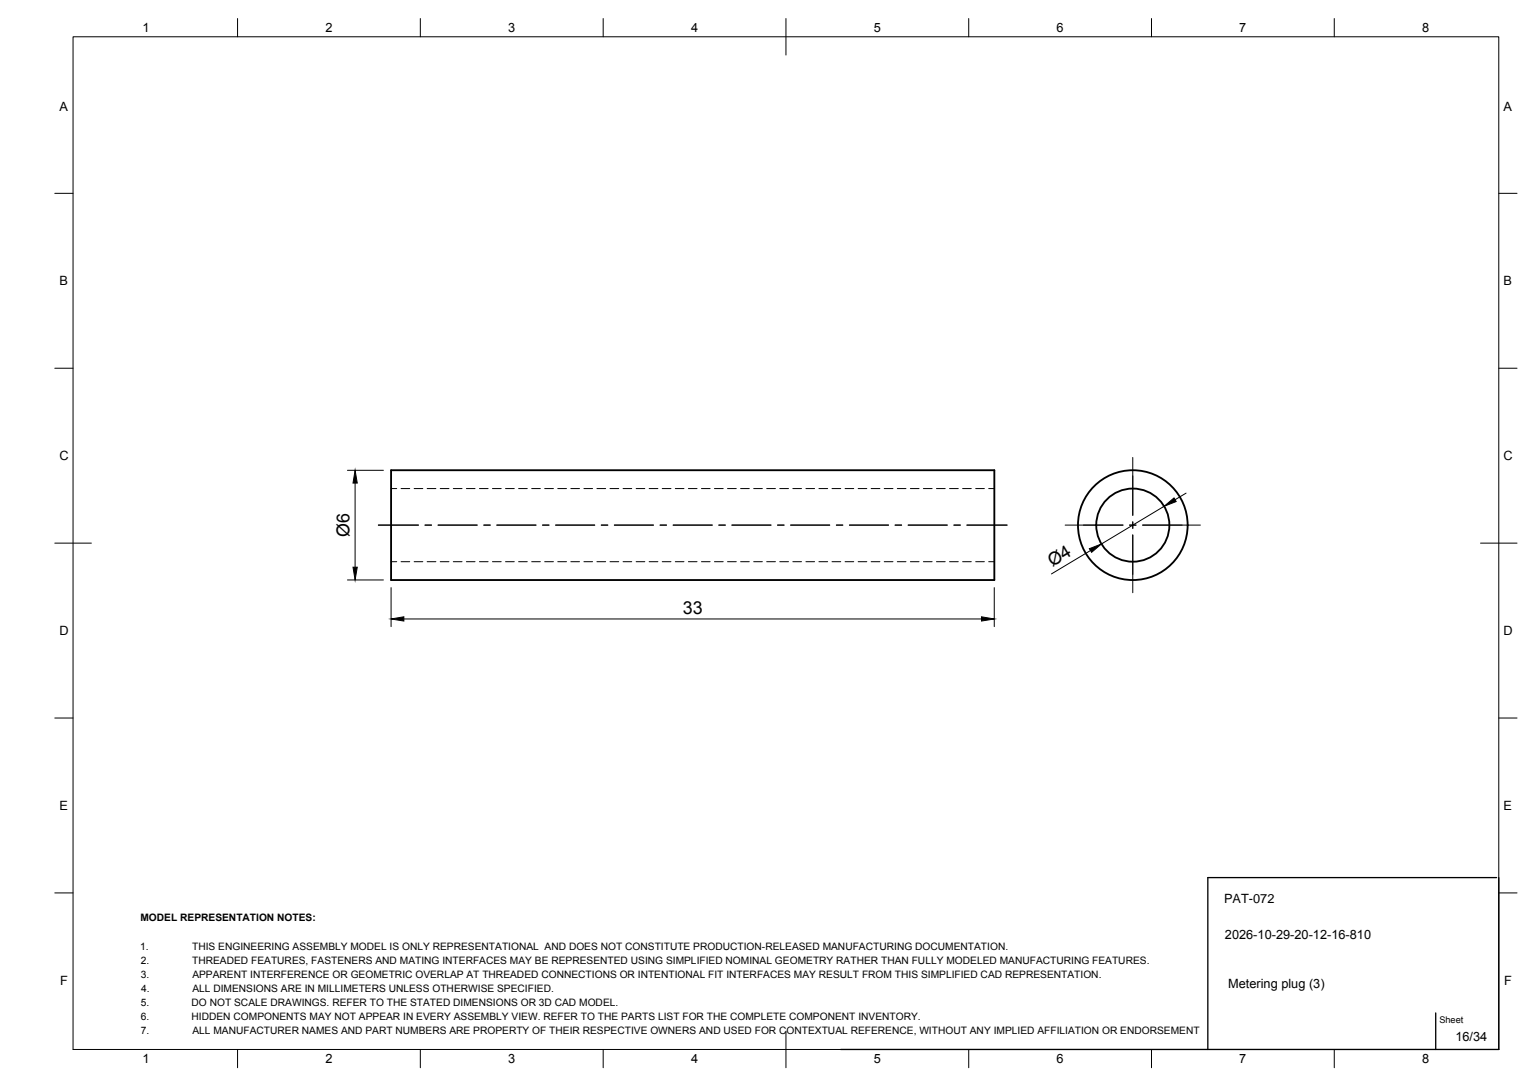
ISO-10303-21;
HEADER;
/* Generated by software containing ST-Developer
 * from STEP Tools, Inc. (www.steptools.com) 
 */

FILE_DESCRIPTION(
/* description */ ('PAT-072'),
/* implementation_level */ '2;1');

FILE_NAME(
/* name */ 'Metering plug (3).step',
/* time_stamp */ '2026-10-29T20:11:56-07:00',
/* author */ (''),
/* organization */ (''),
/* preprocessor_version */ 'ST-DEVELOPER v20.2',
/* originating_system */ 'Autodesk Translation Framework v15.17.0.0',
/* authorisation */ '');

FILE_SCHEMA (('AUTOMOTIVE_DESIGN { 1 0 10303 214 3 1 1 }'));
ENDSEC;

DATA;
#10=MECHANICAL_DESIGN_GEOMETRIC_PRESENTATION_REPRESENTATION('',(#346),#11432);
#274=SHAPE_REPRESENTATION_RELATIONSHIP('SRR','None',#11578,#310);
#310=ADVANCED_BREP_SHAPE_REPRESENTATION('',(#382),#11409);
#346=STYLED_ITEM('',(#11812),#382);
#382=MANIFOLD_SOLID_BREP('Body1',#6081);
#480=FACE_BOUND('',#1393,.T.);
#481=FACE_BOUND('',#1397,.T.);
#647=PLANE('',#6798);
#648=PLANE('',#6803);
#649=PLANE('',#6804);
#650=PLANE('',#6810);
#942=FACE_OUTER_BOUND('',#1392,.T.);
#943=FACE_OUTER_BOUND('',#1394,.T.);
#944=FACE_OUTER_BOUND('',#1395,.T.);
#945=FACE_OUTER_BOUND('',#1396,.T.);
#946=FACE_OUTER_BOUND('',#1398,.T.);
#947=FACE_OUTER_BOUND('',#1399,.T.);
#948=FACE_OUTER_BOUND('',#1400,.T.);
#1392=EDGE_LOOP('',(#4636));
#1393=EDGE_LOOP('',(#4637));
#1394=EDGE_LOOP('',(#4638,#4639,#4640,#4641));
#1395=EDGE_LOOP('',(#4642));
#1396=EDGE_LOOP('',(#4643));
#1397=EDGE_LOOP('',(#4644));
#1398=EDGE_LOOP('',(#4645,#4646,#4647,#4648));
#1399=EDGE_LOOP('',(#4649,#4650,#4651,#4652));
#1400=EDGE_LOOP('',(#4653));
#1833=LINE('',#10171,#2252);
#1834=LINE('',#10179,#2253);
#1835=LINE('',#10182,#2254);
#2252=VECTOR('',#7986,0.6);
#2253=VECTOR('',#7997,0.3);
#2254=VECTOR('',#8000,0.1);
#2673=CIRCLE('',#6799,0.6);
#2674=CIRCLE('',#6800,0.3);
#2675=CIRCLE('',#6802,0.6);
#2676=CIRCLE('',#6805,0.3);
#2677=CIRCLE('',#6806,0.1);
#2678=CIRCLE('',#6809,0.1);
#3022=VERTEX_POINT('',#10164);
#3023=VERTEX_POINT('',#10166);
#3024=VERTEX_POINT('',#10169);
#3025=VERTEX_POINT('',#10174);
#3026=VERTEX_POINT('',#10176);
#3027=VERTEX_POINT('',#10181);
#3607=EDGE_CURVE('',#3022,#3022,#2673,.T.);
#3608=EDGE_CURVE('',#3023,#3023,#2674,.T.);
#3609=EDGE_CURVE('',#3024,#3024,#2675,.T.);
#3610=EDGE_CURVE('',#3024,#3022,#1833,.T.);
#3611=EDGE_CURVE('',#3025,#3025,#2676,.T.);
#3612=EDGE_CURVE('',#3026,#3026,#2677,.T.);
#3613=EDGE_CURVE('',#3023,#3025,#1834,.T.);
#3614=EDGE_CURVE('',#3026,#3027,#1835,.T.);
#3615=EDGE_CURVE('',#3027,#3027,#2678,.T.);
#4636=ORIENTED_EDGE('',*,*,#3607,.F.);
#4637=ORIENTED_EDGE('',*,*,#3608,.T.);
#4638=ORIENTED_EDGE('',*,*,#3609,.F.);
#4639=ORIENTED_EDGE('',*,*,#3610,.T.);
#4640=ORIENTED_EDGE('',*,*,#3607,.T.);
#4641=ORIENTED_EDGE('',*,*,#3610,.F.);
#4642=ORIENTED_EDGE('',*,*,#3609,.T.);
#4643=ORIENTED_EDGE('',*,*,#3611,.F.);
#4644=ORIENTED_EDGE('',*,*,#3612,.T.);
#4645=ORIENTED_EDGE('',*,*,#3608,.F.);
#4646=ORIENTED_EDGE('',*,*,#3613,.T.);
#4647=ORIENTED_EDGE('',*,*,#3611,.T.);
#4648=ORIENTED_EDGE('',*,*,#3613,.F.);
#4649=ORIENTED_EDGE('',*,*,#3612,.F.);
#4650=ORIENTED_EDGE('',*,*,#3614,.T.);
#4651=ORIENTED_EDGE('',*,*,#3615,.T.);
#4652=ORIENTED_EDGE('',*,*,#3614,.F.);
#4653=ORIENTED_EDGE('',*,*,#3615,.F.);
#5627=CYLINDRICAL_SURFACE('',#6801,0.6);
#5628=CYLINDRICAL_SURFACE('',#6807,0.3);
#5629=CYLINDRICAL_SURFACE('',#6808,0.1);
#5841=ADVANCED_FACE('',(#942,#480),#647,.F.);
#5842=ADVANCED_FACE('',(#943),#5627,.T.);
#5843=ADVANCED_FACE('',(#944),#648,.T.);
#5844=ADVANCED_FACE('',(#945,#481),#649,.F.);
#5845=ADVANCED_FACE('',(#946),#5628,.T.);
#5846=ADVANCED_FACE('',(#947),#5629,.T.);
#5847=ADVANCED_FACE('',(#948),#650,.F.);
#6081=CLOSED_SHELL('',(#5841,#5842,#5843,#5844,#5845,#5846,#5847));
#6797=AXIS2_PLACEMENT_3D('',#10162,#7974,#7975);
#6798=AXIS2_PLACEMENT_3D('',#10163,#7976,#7977);
#6799=AXIS2_PLACEMENT_3D('',#10165,#7978,#7979);
#6800=AXIS2_PLACEMENT_3D('',#10167,#7980,#7981);
#6801=AXIS2_PLACEMENT_3D('',#10168,#7982,#7983);
#6802=AXIS2_PLACEMENT_3D('',#10170,#7984,#7985);
#6803=AXIS2_PLACEMENT_3D('',#10172,#7987,#7988);
#6804=AXIS2_PLACEMENT_3D('',#10173,#7989,#7990);
#6805=AXIS2_PLACEMENT_3D('',#10175,#7991,#7992);
#6806=AXIS2_PLACEMENT_3D('',#10177,#7993,#7994);
#6807=AXIS2_PLACEMENT_3D('',#10178,#7995,#7996);
#6808=AXIS2_PLACEMENT_3D('',#10180,#7998,#7999);
#6809=AXIS2_PLACEMENT_3D('',#10183,#8001,#8002);
#6810=AXIS2_PLACEMENT_3D('',#10184,#8003,#8004);
#7974=DIRECTION('axis',(0.,0.,1.));
#7975=DIRECTION('refdir',(1.,0.,0.));
#7976=DIRECTION('center_axis',(0.,0.,1.));
#7977=DIRECTION('ref_axis',(1.,0.,0.));
#7978=DIRECTION('center_axis',(0.,0.,1.));
#7979=DIRECTION('ref_axis',(1.,0.,0.));
#7980=DIRECTION('center_axis',(0.,0.,1.));
#7981=DIRECTION('ref_axis',(1.,0.,0.));
#7982=DIRECTION('center_axis',(0.,0.,1.));
#7983=DIRECTION('ref_axis',(1.,0.,0.));
#7984=DIRECTION('center_axis',(0.,0.,1.));
#7985=DIRECTION('ref_axis',(1.,0.,0.));
#7986=DIRECTION('',(0.,0.,-1.));
#7987=DIRECTION('center_axis',(0.,0.,1.));
#7988=DIRECTION('ref_axis',(1.,0.,0.));
#7989=DIRECTION('center_axis',(0.,0.,1.));
#7990=DIRECTION('ref_axis',(1.,0.,0.));
#7991=DIRECTION('center_axis',(0.,0.,1.));
#7992=DIRECTION('ref_axis',(1.,0.,0.));
#7993=DIRECTION('center_axis',(0.,0.,1.));
#7994=DIRECTION('ref_axis',(1.,0.,0.));
#7995=DIRECTION('center_axis',(0.,0.,1.));
#7996=DIRECTION('ref_axis',(1.,0.,0.));
#7997=DIRECTION('',(0.,0.,-1.));
#7998=DIRECTION('center_axis',(0.,0.,1.));
#7999=DIRECTION('ref_axis',(1.,0.,0.));
#8000=DIRECTION('',(0.,0.,-1.));
#8001=DIRECTION('center_axis',(0.,0.,1.));
#8002=DIRECTION('ref_axis',(1.,0.,0.));
#8003=DIRECTION('center_axis',(0.,0.,1.));
#8004=DIRECTION('ref_axis',(1.,0.,0.));
#10162=CARTESIAN_POINT('',(0.,0.,0.));
#10163=CARTESIAN_POINT('Origin',(3.75,1.5,6.1));
#10164=CARTESIAN_POINT('',(3.15,1.5,6.1));
#10165=CARTESIAN_POINT('Origin',(3.75,1.5,6.1));
#10166=CARTESIAN_POINT('',(3.45,1.5,6.1));
#10167=CARTESIAN_POINT('Origin',(3.75,1.5,6.1));
#10168=CARTESIAN_POINT('Origin',(3.75,1.5,6.1));
#10169=CARTESIAN_POINT('',(3.15,1.5,6.5));
#10170=CARTESIAN_POINT('Origin',(3.75,1.5,6.5));
#10171=CARTESIAN_POINT('',(3.15,1.5,6.1));
#10172=CARTESIAN_POINT('Origin',(3.75,1.5,6.5));
#10173=CARTESIAN_POINT('Origin',(3.75,1.5,4.8));
#10174=CARTESIAN_POINT('',(3.45,1.5,4.8));
#10175=CARTESIAN_POINT('Origin',(3.75,1.5,4.8));
#10176=CARTESIAN_POINT('',(3.65,1.5,4.8));
#10177=CARTESIAN_POINT('Origin',(3.75,1.5,4.8));
#10178=CARTESIAN_POINT('Origin',(3.75,1.5,4.8));
#10179=CARTESIAN_POINT('',(3.45,1.5,4.8));
#10180=CARTESIAN_POINT('Origin',(3.75,1.5,4.1));
#10181=CARTESIAN_POINT('',(3.65,1.5,4.1));
#10182=CARTESIAN_POINT('',(3.65,1.5,4.1));
#10183=CARTESIAN_POINT('Origin',(3.75,1.5,4.1));
#10184=CARTESIAN_POINT('Origin',(3.75,1.5,4.1));
#11370=UNCERTAINTY_MEASURE_WITH_UNIT(LENGTH_MEASURE(0.001),#11433,
'DISTANCE_ACCURACY_VALUE',
'Maximum model space distance between geometric entities at asserted c
onnectivities');
#11393=UNCERTAINTY_MEASURE_WITH_UNIT(LENGTH_MEASURE(0.001),#11433,
'DISTANCE_ACCURACY_VALUE',
'Maximum model space distance between geometric entities at asserted c
onnectivities');
#11409=(
GEOMETRIC_REPRESENTATION_CONTEXT(3)
GLOBAL_UNCERTAINTY_ASSIGNED_CONTEXT((#11370))
GLOBAL_UNIT_ASSIGNED_CONTEXT((#11433,#11435,#11436))
REPRESENTATION_CONTEXT('','3D')
);
#11432=(
GEOMETRIC_REPRESENTATION_CONTEXT(3)
GLOBAL_UNCERTAINTY_ASSIGNED_CONTEXT((#11393))
GLOBAL_UNIT_ASSIGNED_CONTEXT((#11433,#11435,#11436))
REPRESENTATION_CONTEXT('','3D')
);
#11433=(
LENGTH_UNIT()
NAMED_UNIT(*)
SI_UNIT(.CENTI.,.METRE.)
);
#11435=(
NAMED_UNIT(*)
PLANE_ANGLE_UNIT()
SI_UNIT($,.RADIAN.)
);
#11436=(
NAMED_UNIT(*)
SI_UNIT($,.STERADIAN.)
SOLID_ANGLE_UNIT()
);
#11452=SHAPE_DEFINITION_REPRESENTATION(#11490,#11578);
#11490=PRODUCT_DEFINITION_SHAPE('',$,#11617);
#11578=SHAPE_REPRESENTATION('',(#6797),#11409);
#11601=PRODUCT_DEFINITION_CONTEXT('part definition',#11717,'design');
#11617=PRODUCT_DEFINITION('Metering plug (3)',
'Metering plug (3)',#11655,#11601);
#11655=PRODUCT_DEFINITION_FORMATION('',$,#11734);
#11717=APPLICATION_CONTEXT(
'Core Data for Automotive Mechanical Design Process');
#11718=PRODUCT_CONTEXT('part definition',#11717,'mechanical');
#11734=PRODUCT('Metering plug (3)','Metering plug (3)',
'Metering plug (3)',(#11718));
#11806=COLOUR_RGB('Sky Blue',0.24,0.69,0.87);
#11807=FILL_AREA_STYLE_COLOUR('',#11806);
#11808=FILL_AREA_STYLE('',(#11807));
#11809=SURFACE_STYLE_FILL_AREA(#11808);
#11810=SURFACE_SIDE_STYLE('',(#11809));
#11811=SURFACE_STYLE_USAGE(.BOTH.,#11810);
#11812=PRESENTATION_STYLE_ASSIGNMENT((#11811));
ENDSEC;
END-ISO-10303-21;
